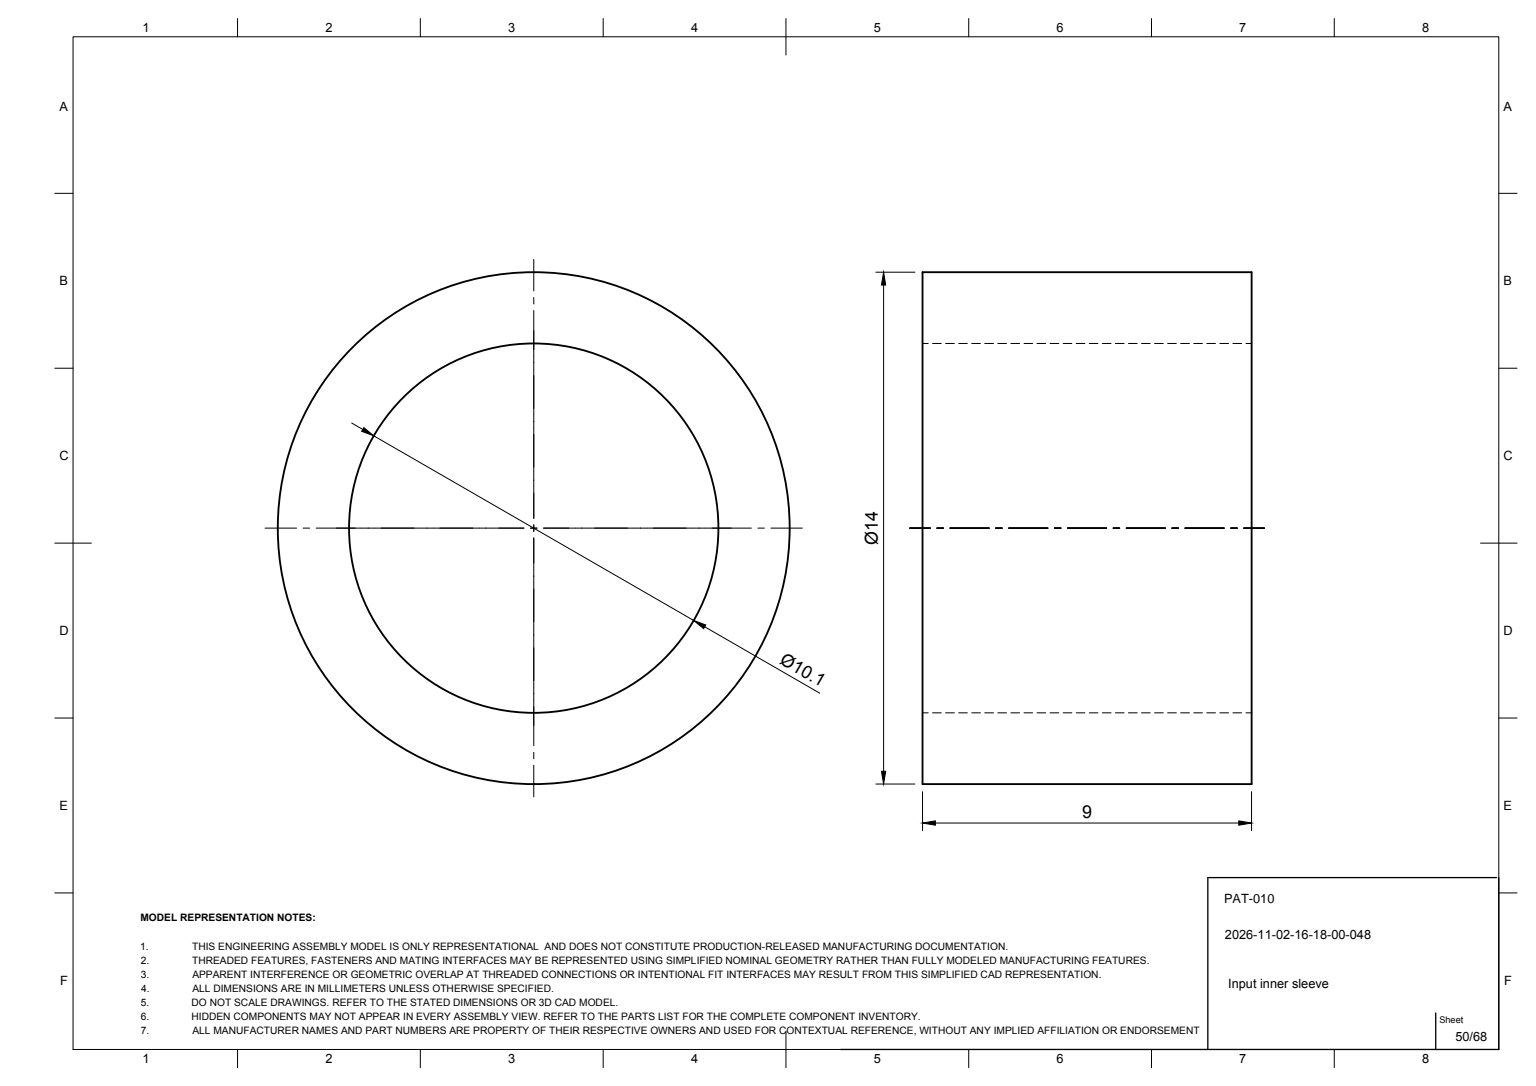
ISO-10303-21;
HEADER;
/* Generated by software containing ST-Developer
 * from STEP Tools, Inc. (www.steptools.com) 
 */

FILE_DESCRIPTION(
/* description */ ('Belt conveyor head drive unit'),
/* implementation_level */ '2;1');

FILE_NAME(
/* name */ 'Input inner sleeve.step',
/* time_stamp */ '2026-10-28T03:26:19-07:00',
/* author */ (''),
/* organization */ (''),
/* preprocessor_version */ 'ST-DEVELOPER v20.2',
/* originating_system */ 'Autodesk Translation Framework v15.17.0.0',
/* authorisation */ '');

FILE_SCHEMA (('AUTOMOTIVE_DESIGN { 1 0 10303 214 3 1 1 }'));
ENDSEC;

DATA;
#10=MECHANICAL_DESIGN_GEOMETRIC_PRESENTATION_REPRESENTATION('',(#909),#27069);
#755=SHAPE_REPRESENTATION_RELATIONSHIP('SRR','None',#27403,#824);
#824=ADVANCED_BREP_SHAPE_REPRESENTATION('',(#990),#27045);
#909=STYLED_ITEM('',(#27783),#990);
#990=MANIFOLD_SOLID_BREP('Body1',#13778);
#1212=FACE_BOUND('',#3167,.T.);
#1213=FACE_BOUND('',#3169,.T.);
#1550=PLANE('',#15679);
#1551=PLANE('',#15680);
#2164=FACE_OUTER_BOUND('',#3164,.T.);
#2165=FACE_OUTER_BOUND('',#3165,.T.);
#2166=FACE_OUTER_BOUND('',#3166,.T.);
#2167=FACE_OUTER_BOUND('',#3168,.T.);
#3164=EDGE_LOOP('',(#11208,#11209,#11210,#11211));
#3165=EDGE_LOOP('',(#11212,#11213,#11214,#11215));
#3166=EDGE_LOOP('',(#11216));
#3167=EDGE_LOOP('',(#11217));
#3168=EDGE_LOOP('',(#11218));
#3169=EDGE_LOOP('',(#11219));
#4052=LINE('',#24505,#4844);
#4053=LINE('',#24511,#4845);
#4844=VECTOR('',#19214,0.505);
#4845=VECTOR('',#19221,0.7);
#5597=CIRCLE('',#15674,0.505);
#5598=CIRCLE('',#15675,0.505);
#5599=CIRCLE('',#15677,0.7);
#5600=CIRCLE('',#15678,0.7);
#6723=VERTEX_POINT('',#24502);
#6724=VERTEX_POINT('',#24504);
#6725=VERTEX_POINT('',#24508);
#6726=VERTEX_POINT('',#24510);
#8296=EDGE_CURVE('',#6723,#6723,#5597,.T.);
#8297=EDGE_CURVE('',#6723,#6724,#4052,.T.);
#8298=EDGE_CURVE('',#6724,#6724,#5598,.T.);
#8299=EDGE_CURVE('',#6725,#6725,#5599,.T.);
#8300=EDGE_CURVE('',#6725,#6726,#4053,.T.);
#8301=EDGE_CURVE('',#6726,#6726,#5600,.T.);
#11208=ORIENTED_EDGE('',*,*,#8296,.F.);
#11209=ORIENTED_EDGE('',*,*,#8297,.T.);
#11210=ORIENTED_EDGE('',*,*,#8298,.T.);
#11211=ORIENTED_EDGE('',*,*,#8297,.F.);
#11212=ORIENTED_EDGE('',*,*,#8299,.F.);
#11213=ORIENTED_EDGE('',*,*,#8300,.T.);
#11214=ORIENTED_EDGE('',*,*,#8301,.T.);
#11215=ORIENTED_EDGE('',*,*,#8300,.F.);
#11216=ORIENTED_EDGE('',*,*,#8299,.T.);
#11217=ORIENTED_EDGE('',*,*,#8296,.T.);
#11218=ORIENTED_EDGE('',*,*,#8301,.F.);
#11219=ORIENTED_EDGE('',*,*,#8298,.F.);
#12732=CYLINDRICAL_SURFACE('',#15673,0.505);
#12733=CYLINDRICAL_SURFACE('',#15676,0.7);
#13443=ADVANCED_FACE('',(#2164),#12732,.F.);
#13444=ADVANCED_FACE('',(#2165),#12733,.T.);
#13445=ADVANCED_FACE('',(#2166,#1212),#1550,.T.);
#13446=ADVANCED_FACE('',(#2167,#1213),#1551,.F.);
#13778=CLOSED_SHELL('',(#13443,#13444,#13445,#13446));
#15672=AXIS2_PLACEMENT_3D('',#24500,#19208,#19209);
#15673=AXIS2_PLACEMENT_3D('',#24501,#19210,#19211);
#15674=AXIS2_PLACEMENT_3D('',#24503,#19212,#19213);
#15675=AXIS2_PLACEMENT_3D('',#24506,#19215,#19216);
#15676=AXIS2_PLACEMENT_3D('',#24507,#19217,#19218);
#15677=AXIS2_PLACEMENT_3D('',#24509,#19219,#19220);
#15678=AXIS2_PLACEMENT_3D('',#24512,#19222,#19223);
#15679=AXIS2_PLACEMENT_3D('',#24513,#19224,#19225);
#15680=AXIS2_PLACEMENT_3D('',#24514,#19226,#19227);
#19208=DIRECTION('axis',(0.,0.,1.));
#19209=DIRECTION('refdir',(1.,0.,0.));
#19210=DIRECTION('center_axis',(0.,1.,0.));
#19211=DIRECTION('ref_axis',(1.,0.,0.));
#19212=DIRECTION('center_axis',(0.,-1.,0.));
#19213=DIRECTION('ref_axis',(1.,0.,0.));
#19214=DIRECTION('',(0.,-1.,0.));
#19215=DIRECTION('center_axis',(0.,-1.,0.));
#19216=DIRECTION('ref_axis',(1.,0.,0.));
#19217=DIRECTION('center_axis',(0.,1.,0.));
#19218=DIRECTION('ref_axis',(1.,0.,0.));
#19219=DIRECTION('center_axis',(0.,1.,0.));
#19220=DIRECTION('ref_axis',(1.,0.,0.));
#19221=DIRECTION('',(0.,-1.,0.));
#19222=DIRECTION('center_axis',(0.,1.,0.));
#19223=DIRECTION('ref_axis',(1.,0.,0.));
#19224=DIRECTION('center_axis',(0.,1.,0.));
#19225=DIRECTION('ref_axis',(1.,0.,0.));
#19226=DIRECTION('center_axis',(0.,1.,0.));
#19227=DIRECTION('ref_axis',(1.,0.,0.));
#24500=CARTESIAN_POINT('',(0.,0.,0.));
#24501=CARTESIAN_POINT('Origin',(0.,-0.45,7.));
#24502=CARTESIAN_POINT('',(-0.505,0.45,7.));
#24503=CARTESIAN_POINT('Origin',(0.,0.45,7.));
#24504=CARTESIAN_POINT('',(-0.505,-0.45,7.));
#24505=CARTESIAN_POINT('',(-0.505,-0.45,7.));
#24506=CARTESIAN_POINT('Origin',(0.,-0.45,7.));
#24507=CARTESIAN_POINT('Origin',(0.,-0.45,7.));
#24508=CARTESIAN_POINT('',(-0.7,0.45,7.));
#24509=CARTESIAN_POINT('Origin',(0.,0.45,7.));
#24510=CARTESIAN_POINT('',(-0.7,-0.45,7.));
#24511=CARTESIAN_POINT('',(-0.7,-0.45,7.));
#24512=CARTESIAN_POINT('Origin',(0.,-0.45,7.));
#24513=CARTESIAN_POINT('Origin',(0.,0.45,7.));
#24514=CARTESIAN_POINT('Origin',(0.,-0.45,7.));
#26968=UNCERTAINTY_MEASURE_WITH_UNIT(LENGTH_MEASURE(0.001),#27070,
'DISTANCE_ACCURACY_VALUE',
'Maximum model space distance between geometric entities at asserted c
onnectivities');
#26992=UNCERTAINTY_MEASURE_WITH_UNIT(LENGTH_MEASURE(0.001),#27070,
'DISTANCE_ACCURACY_VALUE',
'Maximum model space distance between geometric entities at asserted c
onnectivities');
#27045=(
GEOMETRIC_REPRESENTATION_CONTEXT(3)
GLOBAL_UNCERTAINTY_ASSIGNED_CONTEXT((#26968))
GLOBAL_UNIT_ASSIGNED_CONTEXT((#27070,#27072,#27073))
REPRESENTATION_CONTEXT('','3D')
);
#27069=(
GEOMETRIC_REPRESENTATION_CONTEXT(3)
GLOBAL_UNCERTAINTY_ASSIGNED_CONTEXT((#26992))
GLOBAL_UNIT_ASSIGNED_CONTEXT((#27070,#27072,#27073))
REPRESENTATION_CONTEXT('','3D')
);
#27070=(
LENGTH_UNIT()
NAMED_UNIT(*)
SI_UNIT(.CENTI.,.METRE.)
);
#27072=(
NAMED_UNIT(*)
PLANE_ANGLE_UNIT()
SI_UNIT($,.RADIAN.)
);
#27073=(
NAMED_UNIT(*)
SI_UNIT($,.STERADIAN.)
SOLID_ANGLE_UNIT()
);
#27126=SHAPE_DEFINITION_REPRESENTATION(#27214,#27403);
#27214=PRODUCT_DEFINITION_SHAPE('',$,#27480);
#27403=SHAPE_REPRESENTATION('',(#15672),#27045);
#27427=PRODUCT_DEFINITION_CONTEXT('part definition',#27657,'design');
#27480=PRODUCT_DEFINITION('Input inner sleeve','Input inner sleeve',#27556,
#27427);
#27556=PRODUCT_DEFINITION_FORMATION('',$,#27711);
#27657=APPLICATION_CONTEXT(
'Core Data for Automotive Mechanical Design Process');
#27658=PRODUCT_CONTEXT('part definition',#27657,'mechanical');
#27711=PRODUCT('Input inner sleeve','Input inner sleeve',
'Input inner sleeve',(#27658));
#27777=COLOUR_RGB('Light Blue',0.38,0.62,0.78);
#27778=FILL_AREA_STYLE_COLOUR('',#27777);
#27779=FILL_AREA_STYLE('',(#27778));
#27780=SURFACE_STYLE_FILL_AREA(#27779);
#27781=SURFACE_SIDE_STYLE('',(#27780));
#27782=SURFACE_STYLE_USAGE(.BOTH.,#27781);
#27783=PRESENTATION_STYLE_ASSIGNMENT((#27782));
ENDSEC;
END-ISO-10303-21;
